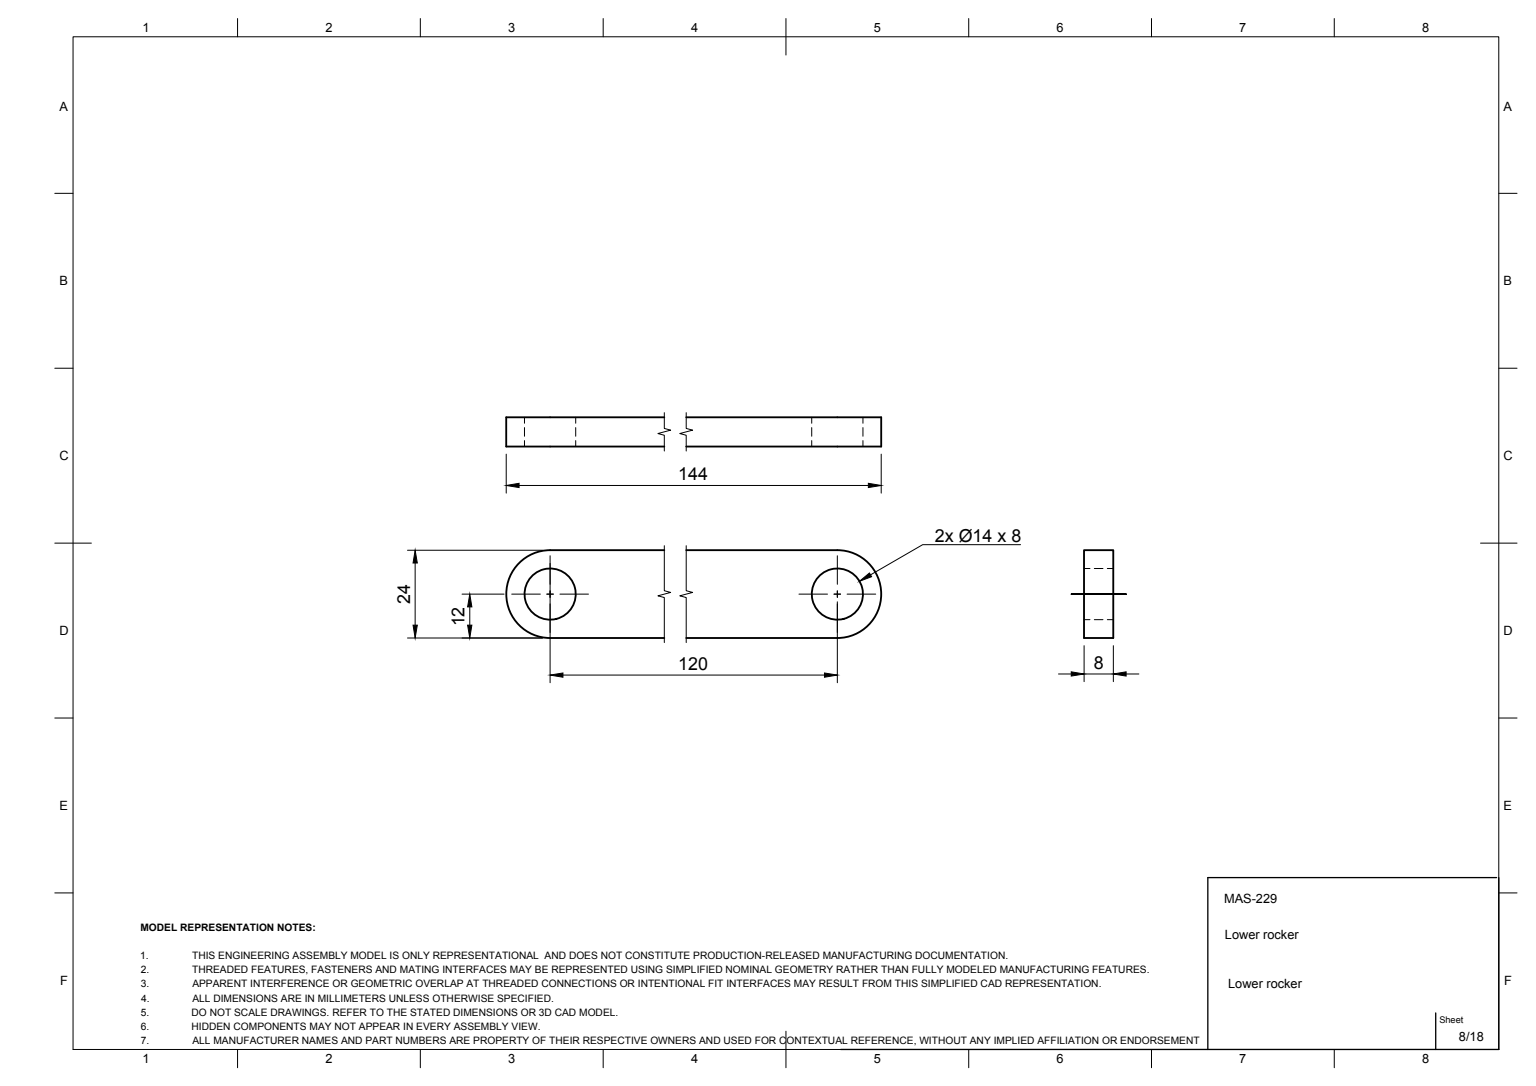
ISO-10303-21;
HEADER;
/* Generated by software containing ST-Developer
 * from STEP Tools, Inc. (www.steptools.com) 
 */

FILE_DESCRIPTION(
/* description */ ('Independently dimensioned six-bar single-leg walking-linkage demonstr
ator. Whole-mm20 crank,60 upper rocker,80/120 ternary coupler,120 lowe
r rocker,140 knee pitch and260 toe reach; ground pivots0/0,60/0,40/60.
 Seven native revolutes close both loops. Four reused native library f
amilies, fully retained shared pins and layered real spacer stacks, bo
nded rubber toe. Benchtop reference mechanism; no complete vehicle, lo
ad, gait stability, adhesive, weld, fit or life rating.'),
/* implementation_level */ '2;1');

FILE_NAME(
/* name */ 'Lower rocker.step',
/* time_stamp */ '2026-11-09T20:33:14-08:00',
/* author */ (''),
/* organization */ (''),
/* preprocessor_version */ 'ST-DEVELOPER v20.2',
/* originating_system */ 'Autodesk Translation Framework v15.17.0.0',
/* authorisation */ '');

FILE_SCHEMA (('AUTOMOTIVE_DESIGN { 1 0 10303 214 3 1 1 }'));
ENDSEC;

DATA;
#10=MECHANICAL_DESIGN_GEOMETRIC_PRESENTATION_REPRESENTATION('',(#260),#4048);
#224=SHAPE_REPRESENTATION_RELATIONSHIP('SRR','None',#4148,#242);
#242=ADVANCED_BREP_SHAPE_REPRESENTATION('',(#278),#4035);
#260=STYLED_ITEM('',(#4247),#278);
#278=MANIFOLD_SOLID_BREP('Body1',#2149);
#319=FACE_BOUND('',#622,.T.);
#320=FACE_BOUND('',#623,.T.);
#321=FACE_BOUND('',#625,.T.);
#322=FACE_BOUND('',#626,.T.);
#374=PLANE('',#2460);
#375=PLANE('',#2464);
#376=PLANE('',#2468);
#377=PLANE('',#2469);
#461=FACE_OUTER_BOUND('',#615,.T.);
#462=FACE_OUTER_BOUND('',#616,.T.);
#463=FACE_OUTER_BOUND('',#617,.T.);
#464=FACE_OUTER_BOUND('',#618,.T.);
#465=FACE_OUTER_BOUND('',#619,.T.);
#466=FACE_OUTER_BOUND('',#620,.T.);
#467=FACE_OUTER_BOUND('',#621,.T.);
#468=FACE_OUTER_BOUND('',#624,.T.);
#615=EDGE_LOOP('',(#1701,#1702,#1703,#1704));
#616=EDGE_LOOP('',(#1705,#1706,#1707,#1708));
#617=EDGE_LOOP('',(#1709,#1710,#1711,#1712));
#618=EDGE_LOOP('',(#1713,#1714,#1715,#1716));
#619=EDGE_LOOP('',(#1717,#1718,#1719,#1720));
#620=EDGE_LOOP('',(#1721,#1722,#1723,#1724));
#621=EDGE_LOOP('',(#1725,#1726,#1727,#1728));
#622=EDGE_LOOP('',(#1729));
#623=EDGE_LOOP('',(#1730));
#624=EDGE_LOOP('',(#1731,#1732,#1733,#1734));
#625=EDGE_LOOP('',(#1735));
#626=EDGE_LOOP('',(#1736));
#792=LINE('',#3653,#917);
#793=LINE('',#3659,#918);
#794=LINE('',#3664,#919);
#795=LINE('',#3666,#920);
#796=LINE('',#3668,#921);
#797=LINE('',#3669,#922);
#798=LINE('',#3675,#923);
#799=LINE('',#3678,#924);
#800=LINE('',#3680,#925);
#801=LINE('',#3681,#926);
#917=VECTOR('',#2929,7.);
#918=VECTOR('',#2936,7.);
#919=VECTOR('',#2941,10.);
#920=VECTOR('',#2942,10.);
#921=VECTOR('',#2943,10.);
#922=VECTOR('',#2944,10.);
#923=VECTOR('',#2951,10.);
#924=VECTOR('',#2954,10.);
#925=VECTOR('',#2955,10.);
#926=VECTOR('',#2956,10.);
#1014=CIRCLE('',#2455,7.);
#1015=CIRCLE('',#2456,7.);
#1016=CIRCLE('',#2458,7.);
#1017=CIRCLE('',#2459,7.);
#1018=CIRCLE('',#2462,12.);
#1019=CIRCLE('',#2463,12.);
#1020=CIRCLE('',#2466,12.);
#1021=CIRCLE('',#2467,12.);
#1160=VERTEX_POINT('',#3650);
#1161=VERTEX_POINT('',#3652);
#1162=VERTEX_POINT('',#3656);
#1163=VERTEX_POINT('',#3658);
#1164=VERTEX_POINT('',#3662);
#1165=VERTEX_POINT('',#3663);
#1166=VERTEX_POINT('',#3665);
#1167=VERTEX_POINT('',#3667);
#1168=VERTEX_POINT('',#3671);
#1169=VERTEX_POINT('',#3673);
#1170=VERTEX_POINT('',#3677);
#1171=VERTEX_POINT('',#3679);
#1354=EDGE_CURVE('',#1160,#1160,#1014,.T.);
#1355=EDGE_CURVE('',#1160,#1161,#792,.T.);
#1356=EDGE_CURVE('',#1161,#1161,#1015,.T.);
#1357=EDGE_CURVE('',#1162,#1162,#1016,.T.);
#1358=EDGE_CURVE('',#1162,#1163,#793,.T.);
#1359=EDGE_CURVE('',#1163,#1163,#1017,.T.);
#1360=EDGE_CURVE('',#1164,#1165,#794,.T.);
#1361=EDGE_CURVE('',#1165,#1166,#795,.T.);
#1362=EDGE_CURVE('',#1167,#1166,#796,.T.);
#1363=EDGE_CURVE('',#1164,#1167,#797,.T.);
#1364=EDGE_CURVE('',#1168,#1164,#1018,.T.);
#1365=EDGE_CURVE('',#1169,#1167,#1019,.T.);
#1366=EDGE_CURVE('',#1168,#1169,#798,.T.);
#1367=EDGE_CURVE('',#1170,#1168,#799,.T.);
#1368=EDGE_CURVE('',#1171,#1169,#800,.T.);
#1369=EDGE_CURVE('',#1170,#1171,#801,.T.);
#1370=EDGE_CURVE('',#1165,#1170,#1020,.T.);
#1371=EDGE_CURVE('',#1166,#1171,#1021,.T.);
#1701=ORIENTED_EDGE('',*,*,#1354,.F.);
#1702=ORIENTED_EDGE('',*,*,#1355,.T.);
#1703=ORIENTED_EDGE('',*,*,#1356,.F.);
#1704=ORIENTED_EDGE('',*,*,#1355,.F.);
#1705=ORIENTED_EDGE('',*,*,#1357,.F.);
#1706=ORIENTED_EDGE('',*,*,#1358,.T.);
#1707=ORIENTED_EDGE('',*,*,#1359,.F.);
#1708=ORIENTED_EDGE('',*,*,#1358,.F.);
#1709=ORIENTED_EDGE('',*,*,#1360,.T.);
#1710=ORIENTED_EDGE('',*,*,#1361,.T.);
#1711=ORIENTED_EDGE('',*,*,#1362,.F.);
#1712=ORIENTED_EDGE('',*,*,#1363,.F.);
#1713=ORIENTED_EDGE('',*,*,#1364,.T.);
#1714=ORIENTED_EDGE('',*,*,#1363,.T.);
#1715=ORIENTED_EDGE('',*,*,#1365,.F.);
#1716=ORIENTED_EDGE('',*,*,#1366,.F.);
#1717=ORIENTED_EDGE('',*,*,#1367,.T.);
#1718=ORIENTED_EDGE('',*,*,#1366,.T.);
#1719=ORIENTED_EDGE('',*,*,#1368,.F.);
#1720=ORIENTED_EDGE('',*,*,#1369,.F.);
#1721=ORIENTED_EDGE('',*,*,#1370,.T.);
#1722=ORIENTED_EDGE('',*,*,#1369,.T.);
#1723=ORIENTED_EDGE('',*,*,#1371,.F.);
#1724=ORIENTED_EDGE('',*,*,#1361,.F.);
#1725=ORIENTED_EDGE('',*,*,#1371,.T.);
#1726=ORIENTED_EDGE('',*,*,#1368,.T.);
#1727=ORIENTED_EDGE('',*,*,#1365,.T.);
#1728=ORIENTED_EDGE('',*,*,#1362,.T.);
#1729=ORIENTED_EDGE('',*,*,#1354,.T.);
#1730=ORIENTED_EDGE('',*,*,#1357,.T.);
#1731=ORIENTED_EDGE('',*,*,#1370,.F.);
#1732=ORIENTED_EDGE('',*,*,#1360,.F.);
#1733=ORIENTED_EDGE('',*,*,#1364,.F.);
#1734=ORIENTED_EDGE('',*,*,#1367,.F.);
#1735=ORIENTED_EDGE('',*,*,#1356,.T.);
#1736=ORIENTED_EDGE('',*,*,#1359,.T.);
#1983=CYLINDRICAL_SURFACE('',#2454,7.);
#1984=CYLINDRICAL_SURFACE('',#2457,7.);
#1985=CYLINDRICAL_SURFACE('',#2461,12.);
#1986=CYLINDRICAL_SURFACE('',#2465,12.);
#2064=ADVANCED_FACE('',(#461),#1983,.F.);
#2065=ADVANCED_FACE('',(#462),#1984,.F.);
#2066=ADVANCED_FACE('',(#463),#374,.T.);
#2067=ADVANCED_FACE('',(#464),#1985,.T.);
#2068=ADVANCED_FACE('',(#465),#375,.T.);
#2069=ADVANCED_FACE('',(#466),#1986,.T.);
#2070=ADVANCED_FACE('',(#467,#319,#320),#376,.T.);
#2071=ADVANCED_FACE('',(#468,#321,#322),#377,.F.);
#2149=CLOSED_SHELL('',(#2064,#2065,#2066,#2067,#2068,#2069,#2070,#2071));
#2453=AXIS2_PLACEMENT_3D('',#3648,#2923,#2924);
#2454=AXIS2_PLACEMENT_3D('',#3649,#2925,#2926);
#2455=AXIS2_PLACEMENT_3D('',#3651,#2927,#2928);
#2456=AXIS2_PLACEMENT_3D('',#3654,#2930,#2931);
#2457=AXIS2_PLACEMENT_3D('',#3655,#2932,#2933);
#2458=AXIS2_PLACEMENT_3D('',#3657,#2934,#2935);
#2459=AXIS2_PLACEMENT_3D('',#3660,#2937,#2938);
#2460=AXIS2_PLACEMENT_3D('',#3661,#2939,#2940);
#2461=AXIS2_PLACEMENT_3D('',#3670,#2945,#2946);
#2462=AXIS2_PLACEMENT_3D('',#3672,#2947,#2948);
#2463=AXIS2_PLACEMENT_3D('',#3674,#2949,#2950);
#2464=AXIS2_PLACEMENT_3D('',#3676,#2952,#2953);
#2465=AXIS2_PLACEMENT_3D('',#3682,#2957,#2958);
#2466=AXIS2_PLACEMENT_3D('',#3683,#2959,#2960);
#2467=AXIS2_PLACEMENT_3D('',#3684,#2961,#2962);
#2468=AXIS2_PLACEMENT_3D('',#3685,#2963,#2964);
#2469=AXIS2_PLACEMENT_3D('',#3686,#2965,#2966);
#2923=DIRECTION('axis',(0.,0.,1.));
#2924=DIRECTION('refdir',(1.,0.,0.));
#2925=DIRECTION('center_axis',(0.,0.,-1.));
#2926=DIRECTION('ref_axis',(1.,0.,0.));
#2927=DIRECTION('center_axis',(0.,0.,-1.));
#2928=DIRECTION('ref_axis',(1.,0.,0.));
#2929=DIRECTION('',(0.,0.,-1.));
#2930=DIRECTION('center_axis',(0.,0.,1.));
#2931=DIRECTION('ref_axis',(1.,0.,0.));
#2932=DIRECTION('center_axis',(0.,0.,-1.));
#2933=DIRECTION('ref_axis',(1.,0.,0.));
#2934=DIRECTION('center_axis',(0.,0.,-1.));
#2935=DIRECTION('ref_axis',(1.,0.,0.));
#2936=DIRECTION('',(0.,0.,-1.));
#2937=DIRECTION('center_axis',(0.,0.,1.));
#2938=DIRECTION('ref_axis',(1.,0.,0.));
#2939=DIRECTION('center_axis',(0.,1.,0.));
#2940=DIRECTION('ref_axis',(-1.,0.,0.));
#2941=DIRECTION('',(-1.,0.,0.));
#2942=DIRECTION('',(0.,0.,1.));
#2943=DIRECTION('',(-1.,0.,0.));
#2944=DIRECTION('',(0.,0.,1.));
#2945=DIRECTION('center_axis',(0.,0.,1.));
#2946=DIRECTION('ref_axis',(0.,-1.,0.));
#2947=DIRECTION('center_axis',(0.,0.,1.));
#2948=DIRECTION('ref_axis',(0.,-1.,0.));
#2949=DIRECTION('center_axis',(0.,0.,1.));
#2950=DIRECTION('ref_axis',(0.,-1.,0.));
#2951=DIRECTION('',(0.,0.,1.));
#2952=DIRECTION('center_axis',(0.,-1.,0.));
#2953=DIRECTION('ref_axis',(1.,0.,0.));
#2954=DIRECTION('',(1.,0.,0.));
#2955=DIRECTION('',(1.,0.,0.));
#2956=DIRECTION('',(0.,0.,1.));
#2957=DIRECTION('center_axis',(0.,0.,1.));
#2958=DIRECTION('ref_axis',(0.,1.,0.));
#2959=DIRECTION('center_axis',(0.,0.,1.));
#2960=DIRECTION('ref_axis',(0.,1.,0.));
#2961=DIRECTION('center_axis',(0.,0.,1.));
#2962=DIRECTION('ref_axis',(0.,1.,0.));
#2963=DIRECTION('center_axis',(0.,0.,1.));
#2964=DIRECTION('ref_axis',(1.,0.,0.));
#2965=DIRECTION('center_axis',(0.,0.,1.));
#2966=DIRECTION('ref_axis',(1.,0.,0.));
#3648=CARTESIAN_POINT('',(0.,0.,0.));
#3649=CARTESIAN_POINT('Origin',(0.,0.,4.));
#3650=CARTESIAN_POINT('',(-7.,8.57252759403147E-16,8.));
#3651=CARTESIAN_POINT('Origin',(0.,0.,8.));
#3652=CARTESIAN_POINT('',(-7.,8.57252759403147E-16,0.));
#3653=CARTESIAN_POINT('',(-7.,8.57252759403147E-16,4.));
#3654=CARTESIAN_POINT('Origin',(0.,0.,0.));
#3655=CARTESIAN_POINT('Origin',(120.,0.,4.));
#3656=CARTESIAN_POINT('',(113.,8.57252759403147E-16,8.));
#3657=CARTESIAN_POINT('Origin',(120.,0.,8.));
#3658=CARTESIAN_POINT('',(113.,8.57252759403147E-16,0.));
#3659=CARTESIAN_POINT('',(113.,8.57252759403147E-16,4.));
#3660=CARTESIAN_POINT('Origin',(120.,0.,0.));
#3661=CARTESIAN_POINT('Origin',(120.,12.,0.));
#3662=CARTESIAN_POINT('',(120.,12.,0.));
#3663=CARTESIAN_POINT('',(0.,12.,0.));
#3664=CARTESIAN_POINT('',(120.,12.,0.));
#3665=CARTESIAN_POINT('',(0.,12.,8.));
#3666=CARTESIAN_POINT('',(0.,12.,0.));
#3667=CARTESIAN_POINT('',(120.,12.,8.));
#3668=CARTESIAN_POINT('',(120.,12.,8.));
#3669=CARTESIAN_POINT('',(120.,12.,0.));
#3670=CARTESIAN_POINT('Origin',(120.,-1.11022302462516E-15,0.));
#3671=CARTESIAN_POINT('',(120.,-12.,0.));
#3672=CARTESIAN_POINT('Origin',(120.,-1.11022302462516E-15,0.));
#3673=CARTESIAN_POINT('',(120.,-12.,8.));
#3674=CARTESIAN_POINT('Origin',(120.,-1.11022302462516E-15,8.));
#3675=CARTESIAN_POINT('',(120.,-12.,0.));
#3676=CARTESIAN_POINT('Origin',(0.,-12.,0.));
#3677=CARTESIAN_POINT('',(-1.46957615897682E-15,-12.,0.));
#3678=CARTESIAN_POINT('',(0.,-12.,0.));
#3679=CARTESIAN_POINT('',(-1.46957615897682E-15,-12.,8.));
#3680=CARTESIAN_POINT('',(0.,-12.,8.));
#3681=CARTESIAN_POINT('',(-1.46957615897682E-15,-12.,0.));
#3682=CARTESIAN_POINT('Origin',(0.,0.,0.));
#3683=CARTESIAN_POINT('Origin',(0.,0.,0.));
#3684=CARTESIAN_POINT('Origin',(0.,0.,8.));
#3685=CARTESIAN_POINT('Origin',(60.,0.,8.));
#3686=CARTESIAN_POINT('Origin',(60.,0.,0.));
#4015=UNCERTAINTY_MEASURE_WITH_UNIT(LENGTH_MEASURE(0.01),#4049,
'DISTANCE_ACCURACY_VALUE',
'Maximum model space distance between geometric entities at asserted c
onnectivities');
#4028=UNCERTAINTY_MEASURE_WITH_UNIT(LENGTH_MEASURE(0.01),#4049,
'DISTANCE_ACCURACY_VALUE',
'Maximum model space distance between geometric entities at asserted c
onnectivities');
#4035=(
GEOMETRIC_REPRESENTATION_CONTEXT(3)
GLOBAL_UNCERTAINTY_ASSIGNED_CONTEXT((#4015))
GLOBAL_UNIT_ASSIGNED_CONTEXT((#4049,#4051,#4052))
REPRESENTATION_CONTEXT('','3D')
);
#4048=(
GEOMETRIC_REPRESENTATION_CONTEXT(3)
GLOBAL_UNCERTAINTY_ASSIGNED_CONTEXT((#4028))
GLOBAL_UNIT_ASSIGNED_CONTEXT((#4049,#4051,#4052))
REPRESENTATION_CONTEXT('','3D')
);
#4049=(
LENGTH_UNIT()
NAMED_UNIT(*)
SI_UNIT(.MILLI.,.METRE.)
);
#4051=(
NAMED_UNIT(*)
PLANE_ANGLE_UNIT()
SI_UNIT($,.RADIAN.)
);
#4052=(
NAMED_UNIT(*)
SI_UNIT($,.STERADIAN.)
SOLID_ANGLE_UNIT()
);
#4059=SHAPE_DEFINITION_REPRESENTATION(#4078,#4148);
#4078=PRODUCT_DEFINITION_SHAPE('',$,#4168);
#4148=SHAPE_REPRESENTATION('',(#2453),#4035);
#4161=PRODUCT_DEFINITION_CONTEXT('part definition',#4220,'design');
#4168=PRODUCT_DEFINITION('Lower rocker','Lower rocker',#4187,#4161);
#4187=PRODUCT_DEFINITION_FORMATION('',$,#4228);
#4220=APPLICATION_CONTEXT(
'Core Data for Automotive Mechanical Design Process');
#4221=PRODUCT_CONTEXT('part definition',#4220,'mechanical');
#4228=PRODUCT('Lower rocker','Lower rocker',$,(#4221));
#4247=PRESENTATION_STYLE_ASSIGNMENT((#4261));
#4261=SURFACE_STYLE_USAGE(.BOTH.,#4275);
#4275=SURFACE_SIDE_STYLE('',(#4289));
#4289=SURFACE_STYLE_FILL_AREA(#4303);
#4303=FILL_AREA_STYLE('Lower rocker finish',(#4317));
#4317=FILL_AREA_STYLE_COLOUR('Lower rocker finish',#4331);
#4331=COLOUR_RGB('Lower rocker finish',0.317647058823529,0.686274509803922,
0.890196078431372);
ENDSEC;
END-ISO-10303-21;
